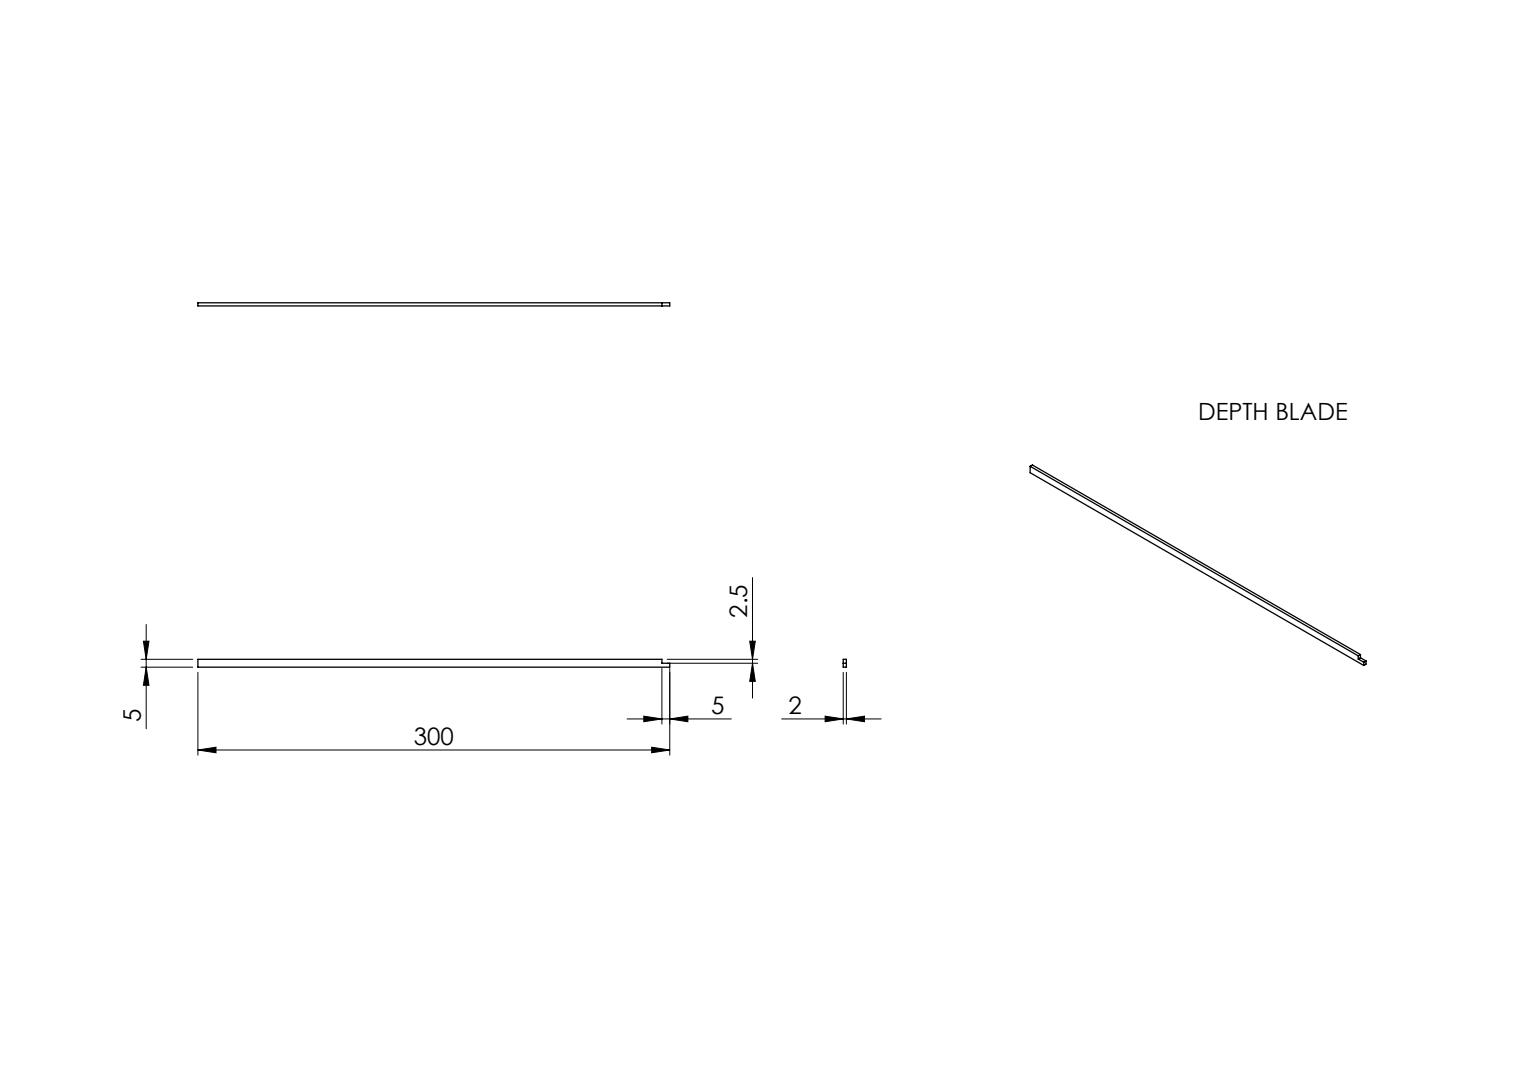
ISO-10303-21;
HEADER;
FILE_DESCRIPTION (('STEP AP214'),
    '1' );
FILE_NAME ('depth blade.step',
    '2026-10-27T04:40:18',
    ( '' ),
    ( '' ),
    'SwSTEP 2.0',
    'SolidWorks 2026',
    '' );
FILE_SCHEMA (( 'AUTOMOTIVE_DESIGN' ));
ENDSEC;

DATA;
#63=ORIENTED_EDGE ( 'NONE', *, *, #6322, .T. ) ;
#97=EDGE_CURVE ( 'NONE', #8537, #7681, #4845, .T. ) ;
#222=AXIS2_PLACEMENT_3D ( 'NONE', #2692, #4339, #10352 ) ;
#275=DIRECTION ( 'NONE',  ( -0.000000000000000000, -1.000000000000000000, -0.000000000000000000 ) ) ;
#326=CARTESIAN_POINT ( 'NONE',  ( 195.0000000000000000, -2.500000000000000000, 2.000000000000000000 ) ) ;
#343=ORIENTED_EDGE ( 'NONE', *, *, #5169, .T. ) ;
#351=( GEOMETRIC_REPRESENTATION_CONTEXT ( 3 ) GLOBAL_UNCERTAINTY_ASSIGNED_CONTEXT ( ( #4611 ) ) GLOBAL_UNIT_ASSIGNED_CONTEXT ( ( #2122, #3664, #4613 ) ) REPRESENTATION_CONTEXT ( 'NONE', 'WORKASPACE' ) );
#431=ORIENTED_EDGE ( 'NONE', *, *, #7584, .F. ) ;
#480=EDGE_LOOP ( 'NONE', ( #9268, #1387, #10634, #9863 ) ) ;
#490=ADVANCED_FACE ( 'NONE', ( #2126 ), #1118, .F. ) ;
#634=PRODUCT_CONTEXT ( 'NONE', #9523, 'mechanical' ) ;
#693=DIRECTION ( 'NONE',  ( 1.000000000000000000, -0.000000000000000000, 0.000000000000000000 ) ) ;
#789=ORIENTED_EDGE ( 'NONE', *, *, #3107, .F. ) ;
#939=PLANE ( 'NONE',  #2806 ) ;
#948=CARTESIAN_POINT ( 'NONE',  ( 195.0000000000000000, -2.500000000000000000, 4.000000000000000000 ) ) ;
#949=CARTESIAN_POINT ( 'NONE',  ( 195.0000000000000000, -2.500000000000000000, 2.000000000000000000 ) ) ;
#961=PLANE ( 'NONE',  #222 ) ;
#1065=DIRECTION ( 'NONE',  ( 0.000000000000000000, 1.000000000000000000, 0.000000000000000000 ) ) ;
#1118=PLANE ( 'NONE',  #10139 ) ;
#1119=VERTEX_POINT ( 'NONE', #3252 ) ;
#1220=AXIS2_PLACEMENT_3D ( 'NONE', #10264, #8446, #2672 ) ;
#1238=AXIS2_PLACEMENT_3D ( 'NONE', #948, #9504, #8510 ) ;
#1262=ADVANCED_FACE ( 'NONE', ( #3631 ), #961, .F. ) ;
#1387=ORIENTED_EDGE ( 'NONE', *, *, #3636, .T. ) ;
#1436=EDGE_LOOP ( 'NONE', ( #3937, #4872, #1658, #9848 ) ) ;
#1457=ADVANCED_FACE ( 'NONE', ( #4571 ), #6535, .T. ) ;
#1485=EDGE_CURVE ( 'NONE', #7100, #1707, #10019, .T. ) ;
#1558=DIRECTION ( 'NONE',  ( 1.000000000000000000, 1.224646799147355672E-16, -0.000000000000000000 ) ) ;
#1598=PRODUCT_DEFINITION_FORMATION_WITH_SPECIFIED_SOURCE ( 'ANY', '', #6542, .NOT_KNOWN. ) ;
#1640=EDGE_LOOP ( 'NONE', ( #7038, #6985, #63, #431, #10351, #8760 ) ) ;
#1658=ORIENTED_EDGE ( 'NONE', *, *, #4363, .T. ) ;
#1706=DIRECTION ( 'NONE',  ( 1.000000000000000000, 0.000000000000000000, 0.000000000000000000 ) ) ;
#1707=VERTEX_POINT ( 'NONE', #949 ) ;
#1759=ORIENTED_EDGE ( 'NONE', *, *, #4363, .F. ) ;
#1802=VECTOR ( 'NONE', #3290, 1000.000000000000000 ) ;
#1824=CARTESIAN_POINT ( 'NONE',  ( -105.0000000000000000, -2.500000000000000000, 4.000000000000000000 ) ) ;
#1837=LINE ( 'NONE', #9282, #10249 ) ;
#1874=CARTESIAN_POINT ( 'NONE',  ( -105.0000000000000000, -2.500000000000000000, 4.000000000000000000 ) ) ;
#1979=CARTESIAN_POINT ( 'NONE',  ( 190.0000000000000000, -6.123233995736783046E-16, 4.000000000000000000 ) ) ;
#2004=CARTESIAN_POINT ( 'NONE',  ( -105.0000000000000000, -2.500000000000000000, 4.000000000000000000 ) ) ;
#2008=VECTOR ( 'NONE', #1065, 1000.000000000000000 ) ;
#2021=EDGE_CURVE ( 'NONE', #8537, #9717, #5962, .T. ) ;
#2046=DIRECTION ( 'NONE',  ( 1.000000000000000000, 0.000000000000000000, 0.000000000000000000 ) ) ;
#2051=CARTESIAN_POINT ( 'NONE',  ( 190.0000000000000000, 0.000000000000000000, 2.000000000000000000 ) ) ;
#2086=DIRECTION ( 'NONE',  ( -1.000000000000000000, 0.000000000000000000, -0.000000000000000000 ) ) ;
#2122=( LENGTH_UNIT ( ) NAMED_UNIT ( * ) SI_UNIT ( .MILLI., .METRE. ) );
#2125=( GEOMETRIC_REPRESENTATION_CONTEXT ( 3 ) GLOBAL_UNCERTAINTY_ASSIGNED_CONTEXT ( ( #5383 ) ) GLOBAL_UNIT_ASSIGNED_CONTEXT ( ( #7766, #2711, #6151 ) ) REPRESENTATION_CONTEXT ( 'NONE', 'WORKASPACE' ) );
#2126=FACE_OUTER_BOUND ( 'NONE', #7599, .T. ) ;
#2238=CARTESIAN_POINT ( 'NONE',  ( 195.0000000000000000, 0.000000000000000000, 4.000000000000000000 ) ) ;
#2307=AXIS2_PLACEMENT_3D ( 'NONE', #5193, #3646, #1706 ) ;
#2490=ORIENTED_EDGE ( 'NONE', *, *, #8209, .T. ) ;
#2531=VECTOR ( 'NONE', #3293, 1000.000000000000000 ) ;
#2537=ORIENTED_EDGE ( 'NONE', *, *, #5651, .F. ) ;
#2556=DIRECTION ( 'NONE',  ( 0.000000000000000000, 0.000000000000000000, -1.000000000000000000 ) ) ;
#2649=COLOUR_RGB ( '',0.8941176470588234615, 0.8941176470588234615, 0.8941176470588234615 ) ;
#2672=DIRECTION ( 'NONE',  ( 0.000000000000000000, -0.000000000000000000, -1.000000000000000000 ) ) ;
#2686=ORIENTED_EDGE ( 'NONE', *, *, #3107, .T. ) ;
#2692=CARTESIAN_POINT ( 'NONE',  ( -105.0000000000000000, -2.500000000000000000, 4.000000000000000000 ) ) ;
#2711=( NAMED_UNIT ( * ) PLANE_ANGLE_UNIT ( ) SI_UNIT ( $, .RADIAN. ) );
#2764=PRESENTATION_STYLE_ASSIGNMENT (( #5139 ) ) ;
#2806=AXIS2_PLACEMENT_3D ( 'NONE', #6053, #5943, #2556 ) ;
#2810=CARTESIAN_POINT ( 'NONE',  ( 195.0000000000000000, -2.500000000000000000, 4.000000000000000000 ) ) ;
#2816=( GEOMETRIC_REPRESENTATION_CONTEXT ( 3 ) GLOBAL_UNCERTAINTY_ASSIGNED_CONTEXT ( ( #6289 ) ) GLOBAL_UNIT_ASSIGNED_CONTEXT ( ( #4680, #9684, #5449 ) ) REPRESENTATION_CONTEXT ( 'NONE', 'WORKASPACE' ) );
#2906=DIRECTION ( 'NONE',  ( 0.000000000000000000, 0.000000000000000000, -1.000000000000000000 ) ) ;
#2930=LINE ( 'NONE', #9699, #3413 ) ;
#2980=EDGE_CURVE ( 'NONE', #8205, #6709, #3997, .T. ) ;
#3043=FACE_OUTER_BOUND ( 'NONE', #480, .T. ) ;
#3107=EDGE_CURVE ( 'NONE', #8537, #8097, #10412, .T. ) ;
#3130=EDGE_CURVE ( 'NONE', #9717, #4004, #7034, .T. ) ;
#3189=EDGE_CURVE ( 'NONE', #4004, #7100, #8044, .T. ) ;
#3252=CARTESIAN_POINT ( 'NONE',  ( 190.0000000000000000, -6.123233995736783046E-16, 2.000000000000000000 ) ) ;
#3290=DIRECTION ( 'NONE',  ( -1.000000000000000000, -0.000000000000000000, -0.000000000000000000 ) ) ;
#3293=DIRECTION ( 'NONE',  ( 1.000000000000000000, 0.000000000000000000, 0.000000000000000000 ) ) ;
#3368=EDGE_LOOP ( 'NONE', ( #7000, #1759, #7052, #8881 ) ) ;
#3370=ORIENTED_EDGE ( 'NONE', *, *, #3130, .T. ) ;
#3413=VECTOR ( 'NONE', #8872, 1000.000000000000000 ) ;
#3533=SURFACE_SIDE_STYLE ('',( #6096 ) ) ;
#3573=EDGE_CURVE ( 'NONE', #9658, #7100, #10738, .T. ) ;
#3587=CARTESIAN_POINT ( 'NONE',  ( 195.0000000000000000, 0.000000000000000000, 4.000000000000000000 ) ) ;
#3602=VECTOR ( 'NONE', #6565, 1000.000000000000000 ) ;
#3606=PLANE ( 'NONE',  #1220 ) ;
#3631=FACE_OUTER_BOUND ( 'NONE', #3368, .T. ) ;
#3636=EDGE_CURVE ( 'NONE', #8097, #8205, #8243, .T. ) ;
#3637=DIRECTION ( 'NONE',  ( -0.000000000000000000, -1.000000000000000000, -0.000000000000000000 ) ) ;
#3646=DIRECTION ( 'NONE',  ( 0.000000000000000000, 0.000000000000000000, 1.000000000000000000 ) ) ;
#3664=( NAMED_UNIT ( * ) PLANE_ANGLE_UNIT ( ) SI_UNIT ( $, .RADIAN. ) );
#3708=DIRECTION ( 'NONE',  ( 0.000000000000000000, -1.000000000000000000, 0.000000000000000000 ) ) ;
#3773=ORIENTED_EDGE ( 'NONE', *, *, #3573, .F. ) ;
#3911=EDGE_LOOP ( 'NONE', ( #7689, #2686, #343, #4233 ) ) ;
#3914=DIRECTION ( 'NONE',  ( -0.000000000000000000, -0.000000000000000000, -1.000000000000000000 ) ) ;
#3937=ORIENTED_EDGE ( 'NONE', *, *, #2980, .F. ) ;
#3959=CARTESIAN_POINT ( 'NONE',  ( -105.0000000000000000, -2.500000000000000000, 4.000000000000000000 ) ) ;
#3979=DIRECTION ( 'NONE',  ( 0.000000000000000000, 0.000000000000000000, -1.000000000000000000 ) ) ;
#3997=LINE ( 'NONE', #10969, #3602 ) ;
#4004=VERTEX_POINT ( 'NONE', #5314 ) ;
#4023=CARTESIAN_POINT ( 'NONE',  ( 195.0000000000000000, -2.500000000000000000, 4.000000000000000000 ) ) ;
#4047=MECHANICAL_DESIGN_GEOMETRIC_PRESENTATION_REPRESENTATION('',(#5815),#2816);
#4076=FACE_OUTER_BOUND ( 'NONE', #3911, .T. ) ;
#4140=CARTESIAN_POINT ( 'NONE',  ( 190.0000000000000000, 2.500000000000000000, 4.000000000000000000 ) ) ;
#4192=VERTEX_POINT ( 'NONE', #2810 ) ;
#4233=ORIENTED_EDGE ( 'NONE', *, *, #9765, .F. ) ;
#4234=STYLED_ITEM ( 'NONE', ( #2764 ), #4690 ) ;
#4326=ORIENTED_EDGE ( 'NONE', *, *, #4701, .T. ) ;
#4339=DIRECTION ( 'NONE',  ( 0.000000000000000000, 1.000000000000000000, 0.000000000000000000 ) ) ;
#4363=EDGE_CURVE ( 'NONE', #4192, #1707, #2930, .T. ) ;
#4370=FACE_OUTER_BOUND ( 'NONE', #6426, .T. ) ;
#4424=VECTOR ( 'NONE', #8004, 1000.000000000000000 ) ;
#4519=ADVANCED_FACE ( 'NONE', ( #4076 ), #9140, .T. ) ;
#4531=LINE ( 'NONE', #1874, #7763 ) ;
#4571=FACE_OUTER_BOUND ( 'NONE', #1640, .T. ) ;
#4583=VECTOR ( 'NONE', #275, 1000.000000000000000 ) ;
#4601=LINE ( 'NONE', #326, #4424 ) ;
#4611=UNCERTAINTY_MEASURE_WITH_UNIT (LENGTH_MEASURE( 1.000000000000000082E-05 ), #2122, 'distance_accuracy_value', 'NONE');
#4613=( NAMED_UNIT ( * ) SI_UNIT ( $, .STERADIAN. ) SOLID_ANGLE_UNIT ( ) );
#4666=VECTOR ( 'NONE', #6917, 1000.000000000000000 ) ;
#4680=( LENGTH_UNIT ( ) NAMED_UNIT ( * ) SI_UNIT ( .MILLI., .METRE. ) );
#4690=ADVANCED_BREP_SHAPE_REPRESENTATION ( '', ( #4847, #2307 ), #351 ) ;
#4701=EDGE_CURVE ( 'NONE', #4192, #8205, #4854, .T. ) ;
#4845=LINE ( 'NONE', #5002, #1802 ) ;
#4847=MANIFOLD_SOLID_BREP ( 'Cut-Extrude1', #10505 ) ;
#4854=LINE ( 'NONE', #4023, #2008 ) ;
#4872=ORIENTED_EDGE ( 'NONE', *, *, #4701, .F. ) ;
#4898=CARTESIAN_POINT ( 'NONE',  ( -105.0000000000000000, -2.500000000000000000, 2.000000000000000000 ) ) ;
#4957=VECTOR ( 'NONE', #7650, 1000.000000000000000 ) ;
#5002=CARTESIAN_POINT ( 'NONE',  ( -105.0000000000000000, 2.500000000000000000, 4.000000000000000000 ) ) ;
#5037=ADVANCED_FACE ( 'NONE', ( #7616 ), #3606, .F. ) ;
#5139=SURFACE_STYLE_USAGE ( .BOTH. , #3533 ) ;
#5169=EDGE_CURVE ( 'NONE', #8097, #1119, #1837, .T. ) ;
#5193=CARTESIAN_POINT ( 'NONE',  ( 0.000000000000000000, 0.000000000000000000, 0.000000000000000000 ) ) ;
#5314=CARTESIAN_POINT ( 'NONE',  ( -105.0000000000000000, 2.500000000000000000, 2.000000000000000000 ) ) ;
#5383=UNCERTAINTY_MEASURE_WITH_UNIT (LENGTH_MEASURE( 1.000000000000000082E-05 ), #7766, 'distance_accuracy_value', 'NONE');
#5404=DIRECTION ( 'NONE',  ( 0.000000000000000000, 0.000000000000000000, -1.000000000000000000 ) ) ;
#5422=EDGE_CURVE ( 'NONE', #7681, #9658, #7896, .T. ) ;
#5449=( NAMED_UNIT ( * ) SI_UNIT ( $, .STERADIAN. ) SOLID_ANGLE_UNIT ( ) );
#5478=VECTOR ( 'NONE', #3914, 1000.000000000000000 ) ;
#5503=CARTESIAN_POINT ( 'NONE',  ( 0.000000000000000000, 0.000000000000000000, 4.000000000000000000 ) ) ;
#5651=EDGE_CURVE ( 'NONE', #7681, #4004, #7410, .T. ) ;
#5723=PRODUCT_DEFINITION_SHAPE ( 'NONE', 'NONE',  #6528 ) ;
#5800=SHAPE_REPRESENTATION ( 'depth blade', ( #2307 ), #351 ) ;
#5815=STYLED_ITEM('',(#11034),#4847);
#5942=DIRECTION ( 'NONE',  ( 0.000000000000000000, 0.000000000000000000, -1.000000000000000000 ) ) ;
#5943=DIRECTION ( 'NONE',  ( 1.000000000000000000, 0.000000000000000000, 0.000000000000000000 ) ) ;
#5962=LINE ( 'NONE', #6133, #4666 ) ;
#6053=CARTESIAN_POINT ( 'NONE',  ( -105.0000000000000000, -2.500000000000000000, 4.000000000000000000 ) ) ;
#6096=SURFACE_STYLE_FILL_AREA ( #10368 ) ;
#6118=PLANE ( 'NONE',  #1238 ) ;
#6133=CARTESIAN_POINT ( 'NONE',  ( 190.0000000000000000, 2.500000000000000000, 4.000000000000000000 ) ) ;
#6151=( NAMED_UNIT ( * ) SI_UNIT ( $, .STERADIAN. ) SOLID_ANGLE_UNIT ( ) );
#6209=APPLICATION_CONTEXT ( 'automotive_design' ) ;
#6218=CARTESIAN_POINT ( 'NONE',  ( 190.0000000000000000, 2.500000000000000000, 2.000000000000000000 ) ) ;
#6246=AXIS2_PLACEMENT_3D ( 'NONE', #8414, #693, #3979 ) ;
#6262=DIRECTION ( 'NONE',  ( -1.000000000000000000, -0.000000000000000000, -0.000000000000000000 ) ) ;
#6265=VECTOR ( 'NONE', #3637, 1000.000000000000000 ) ;
#6289=UNCERTAINTY_MEASURE_WITH_UNIT (LENGTH_MEASURE( 1.000000000000000082E-05 ), #4680, 'distance_accuracy_value', 'NONE');
#6322=EDGE_CURVE ( 'NONE', #1119, #6709, #10136, .T. ) ;
#6346=EDGE_LOOP ( 'NONE', ( #10977, #6470, #3370, #2537 ) ) ;
#6426=EDGE_LOOP ( 'NONE', ( #7938, #3773, #9056, #6573 ) ) ;
#6447=VECTOR ( 'NONE', #10683, 1000.000000000000000 ) ;
#6470=ORIENTED_EDGE ( 'NONE', *, *, #2021, .T. ) ;
#6492=PRODUCT_DEFINITION_CONTEXT ( 'detailed design', #6209, 'design' ) ;
#6528=PRODUCT_DEFINITION ( 'UNKNOWN', '', #1598, #6492 ) ;
#6535=PLANE ( 'NONE',  #10708 ) ;
#6542=PRODUCT ( 'depth blade', 'depth blade', '', ( #634 ) ) ;
#6565=DIRECTION ( 'NONE',  ( 0.000000000000000000, 0.000000000000000000, -1.000000000000000000 ) ) ;
#6573=ORIENTED_EDGE ( 'NONE', *, *, #5651, .T. ) ;
#6636=SHAPE_DEFINITION_REPRESENTATION ( #5723, #5800 ) ;
#6709=VERTEX_POINT ( 'NONE', #8200 ) ;
#6905=ADVANCED_FACE ( 'NONE', ( #7682 ), #6118, .F. ) ;
#6917=DIRECTION ( 'NONE',  ( 0.000000000000000000, 0.000000000000000000, -1.000000000000000000 ) ) ;
#6960=VECTOR ( 'NONE', #1558, 1000.000000000000000 ) ;
#6985=ORIENTED_EDGE ( 'NONE', *, *, #9765, .T. ) ;
#7000=ORIENTED_EDGE ( 'NONE', *, *, #1485, .T. ) ;
#7034=LINE ( 'NONE', #7986, #10318 ) ;
#7038=ORIENTED_EDGE ( 'NONE', *, *, #3130, .F. ) ;
#7052=ORIENTED_EDGE ( 'NONE', *, *, #8209, .F. ) ;
#7100=VERTEX_POINT ( 'NONE', #10565 ) ;
#7248=CARTESIAN_POINT ( 'NONE',  ( -105.0000000000000000, 2.500000000000000000, 4.000000000000000000 ) ) ;
#7410=LINE ( 'NONE', #7248, #5478 ) ;
#7442=MECHANICAL_DESIGN_GEOMETRIC_PRESENTATION_REPRESENTATION('',(#4234),#2125);
#7544=CARTESIAN_POINT ( 'NONE',  ( 190.0000000000000000, -6.123233995736783046E-16, 4.000000000000000000 ) ) ;
#7565=CARTESIAN_POINT ( 'NONE',  ( 195.0000000000000000, 0.000000000000000000, 4.000000000000000000 ) ) ;
#7584=EDGE_CURVE ( 'NONE', #1707, #6709, #4601, .T. ) ;
#7599=EDGE_LOOP ( 'NONE', ( #789, #10703, #8237, #2490, #4326, #8660 ) ) ;
#7602=VECTOR ( 'NONE', #3708, 1000.000000000000000 ) ;
#7616=FACE_OUTER_BOUND ( 'NONE', #6346, .T. ) ;
#7650=DIRECTION ( 'NONE',  ( 1.000000000000000000, 1.224646799147355672E-16, 0.000000000000000000 ) ) ;
#7681=VERTEX_POINT ( 'NONE', #10552 ) ;
#7682=FACE_OUTER_BOUND ( 'NONE', #1436, .T. ) ;
#7689=ORIENTED_EDGE ( 'NONE', *, *, #2021, .F. ) ;
#7763=VECTOR ( 'NONE', #2046, 1000.000000000000000 ) ;
#7766=( LENGTH_UNIT ( ) NAMED_UNIT ( * ) SI_UNIT ( .MILLI., .METRE. ) );
#7896=LINE ( 'NONE', #2004, #4583 ) ;
#7938=ORIENTED_EDGE ( 'NONE', *, *, #3189, .T. ) ;
#7978=CARTESIAN_POINT ( 'NONE',  ( 0.000000000000000000, 0.000000000000000000, 2.000000000000000000 ) ) ;
#7986=CARTESIAN_POINT ( 'NONE',  ( -105.0000000000000000, 2.500000000000000000, 2.000000000000000000 ) ) ;
#8004=DIRECTION ( 'NONE',  ( 0.000000000000000000, 1.000000000000000000, 0.000000000000000000 ) ) ;
#8044=LINE ( 'NONE', #10534, #9099 ) ;
#8097=VERTEX_POINT ( 'NONE', #7544 ) ;
#8200=CARTESIAN_POINT ( 'NONE',  ( 195.0000000000000000, -4.336808689942017736E-16, 2.000000000000000000 ) ) ;
#8205=VERTEX_POINT ( 'NONE', #3587 ) ;
#8209=EDGE_CURVE ( 'NONE', #9658, #4192, #4531, .T. ) ;
#8237=ORIENTED_EDGE ( 'NONE', *, *, #5422, .T. ) ;
#8243=LINE ( 'NONE', #2238, #6960 ) ;
#8414=CARTESIAN_POINT ( 'NONE',  ( 190.0000000000000000, -6.123233995736783046E-16, 4.000000000000000000 ) ) ;
#8446=DIRECTION ( 'NONE',  ( 0.000000000000000000, -1.000000000000000000, 0.000000000000000000 ) ) ;
#8494=AXIS2_PLACEMENT_3D ( 'NONE', #7565, #10844, #10588 ) ;
#8510=DIRECTION ( 'NONE',  ( 0.000000000000000000, 0.000000000000000000, 1.000000000000000000 ) ) ;
#8537=VERTEX_POINT ( 'NONE', #4140 ) ;
#8641=DIRECTION ( 'NONE',  ( -0.000000000000000000, -1.000000000000000000, -0.000000000000000000 ) ) ;
#8660=ORIENTED_EDGE ( 'NONE', *, *, #3636, .F. ) ;
#8760=ORIENTED_EDGE ( 'NONE', *, *, #3189, .F. ) ;
#8872=DIRECTION ( 'NONE',  ( -0.000000000000000000, -0.000000000000000000, -1.000000000000000000 ) ) ;
#8881=ORIENTED_EDGE ( 'NONE', *, *, #3573, .T. ) ;
#9056=ORIENTED_EDGE ( 'NONE', *, *, #5422, .F. ) ;
#9099=VECTOR ( 'NONE', #8641, 1000.000000000000000 ) ;
#9140=PLANE ( 'NONE',  #6246 ) ;
#9151=ADVANCED_FACE ( 'NONE', ( #4370 ), #939, .F. ) ;
#9268=ORIENTED_EDGE ( 'NONE', *, *, #5169, .F. ) ;
#9282=CARTESIAN_POINT ( 'NONE',  ( 190.0000000000000000, -6.123233995736783046E-16, 4.000000000000000000 ) ) ;
#9504=DIRECTION ( 'NONE',  ( -1.000000000000000000, 0.000000000000000000, 0.000000000000000000 ) ) ;
#9523=APPLICATION_CONTEXT ( 'automotive_design' ) ;
#9658=VERTEX_POINT ( 'NONE', #1824 ) ;
#9684=( NAMED_UNIT ( * ) PLANE_ANGLE_UNIT ( ) SI_UNIT ( $, .RADIAN. ) );
#9699=CARTESIAN_POINT ( 'NONE',  ( 195.0000000000000000, -2.500000000000000000, 4.000000000000000000 ) ) ;
#9717=VERTEX_POINT ( 'NONE', #6218 ) ;
#9765=EDGE_CURVE ( 'NONE', #9717, #1119, #10547, .T. ) ;
#9848=ORIENTED_EDGE ( 'NONE', *, *, #7584, .T. ) ;
#9863=ORIENTED_EDGE ( 'NONE', *, *, #6322, .F. ) ;
#10012=PLANE ( 'NONE',  #8494 ) ;
#10019=LINE ( 'NONE', #4898, #2531 ) ;
#10036=CARTESIAN_POINT ( 'NONE',  ( 2.924531576190634356E-30, -2.388061258337343593E-14, 2.000000000000000000 ) ) ;
#10136=LINE ( 'NONE', #10036, #4957 ) ;
#10139=AXIS2_PLACEMENT_3D ( 'NONE', #5503, #2906, #10508 ) ;
#10196=SHAPE_REPRESENTATION_RELATIONSHIP ( 'NONE' , 'NONE' ,  #5800, #4690 ) ;
#10248=FILL_AREA_STYLE_COLOUR ( '', #2649 ) ;
#10249=VECTOR ( 'NONE', #5942, 1000.000000000000000 ) ;
#10264=CARTESIAN_POINT ( 'NONE',  ( -105.0000000000000000, 2.500000000000000000, 4.000000000000000000 ) ) ;
#10318=VECTOR ( 'NONE', #6262, 1000.000000000000000 ) ;
#10351=ORIENTED_EDGE ( 'NONE', *, *, #1485, .F. ) ;
#10352=DIRECTION ( 'NONE',  ( 0.000000000000000000, -0.000000000000000000, 1.000000000000000000 ) ) ;
#10368=FILL_AREA_STYLE ('',( #10248 ) ) ;
#10412=LINE ( 'NONE', #1979, #6265 ) ;
#10483=ADVANCED_FACE ( 'NONE', ( #3043 ), #10012, .T. ) ;
#10505=CLOSED_SHELL ( 'NONE', ( #6905, #490, #1457, #5037, #9151, #1262, #4519, #10483 ) ) ;
#10508=DIRECTION ( 'NONE',  ( -1.000000000000000000, 0.000000000000000000, -0.000000000000000000 ) ) ;
#10534=CARTESIAN_POINT ( 'NONE',  ( -105.0000000000000000, -2.500000000000000000, 2.000000000000000000 ) ) ;
#10547=LINE ( 'NONE', #2051, #7602 ) ;
#10552=CARTESIAN_POINT ( 'NONE',  ( -105.0000000000000000, 2.500000000000000000, 4.000000000000000000 ) ) ;
#10565=CARTESIAN_POINT ( 'NONE',  ( -105.0000000000000000, -2.500000000000000000, 2.000000000000000000 ) ) ;
#10588=DIRECTION ( 'NONE',  ( -1.000000000000000000, -1.224646799147355672E-16, 0.000000000000000000 ) ) ;
#10634=ORIENTED_EDGE ( 'NONE', *, *, #2980, .T. ) ;
#10683=DIRECTION ( 'NONE',  ( -0.000000000000000000, -0.000000000000000000, -1.000000000000000000 ) ) ;
#10703=ORIENTED_EDGE ( 'NONE', *, *, #97, .T. ) ;
#10708=AXIS2_PLACEMENT_3D ( 'NONE', #7978, #5404, #2086 ) ;
#10738=LINE ( 'NONE', #3959, #6447 ) ;
#10844=DIRECTION ( 'NONE',  ( -1.224646799147355672E-16, 1.000000000000000000, 0.000000000000000000 ) ) ;
#10969=CARTESIAN_POINT ( 'NONE',  ( 195.0000000000000000, 0.000000000000000000, 4.000000000000000000 ) ) ;
#10977=ORIENTED_EDGE ( 'NONE', *, *, #97, .F. ) ;
#11028=COLOUR_RGB('Off White',0.89,0.88,0.83);
#11029=FILL_AREA_STYLE_COLOUR('',#11028);
#11030=FILL_AREA_STYLE('',(#11029));
#11031=SURFACE_STYLE_FILL_AREA(#11030);
#11032=SURFACE_SIDE_STYLE('',(#11031));
#11033=SURFACE_STYLE_USAGE(.BOTH.,#11032);
#11034=PRESENTATION_STYLE_ASSIGNMENT((#11033));
ENDSEC;
END-ISO-10303-21;
